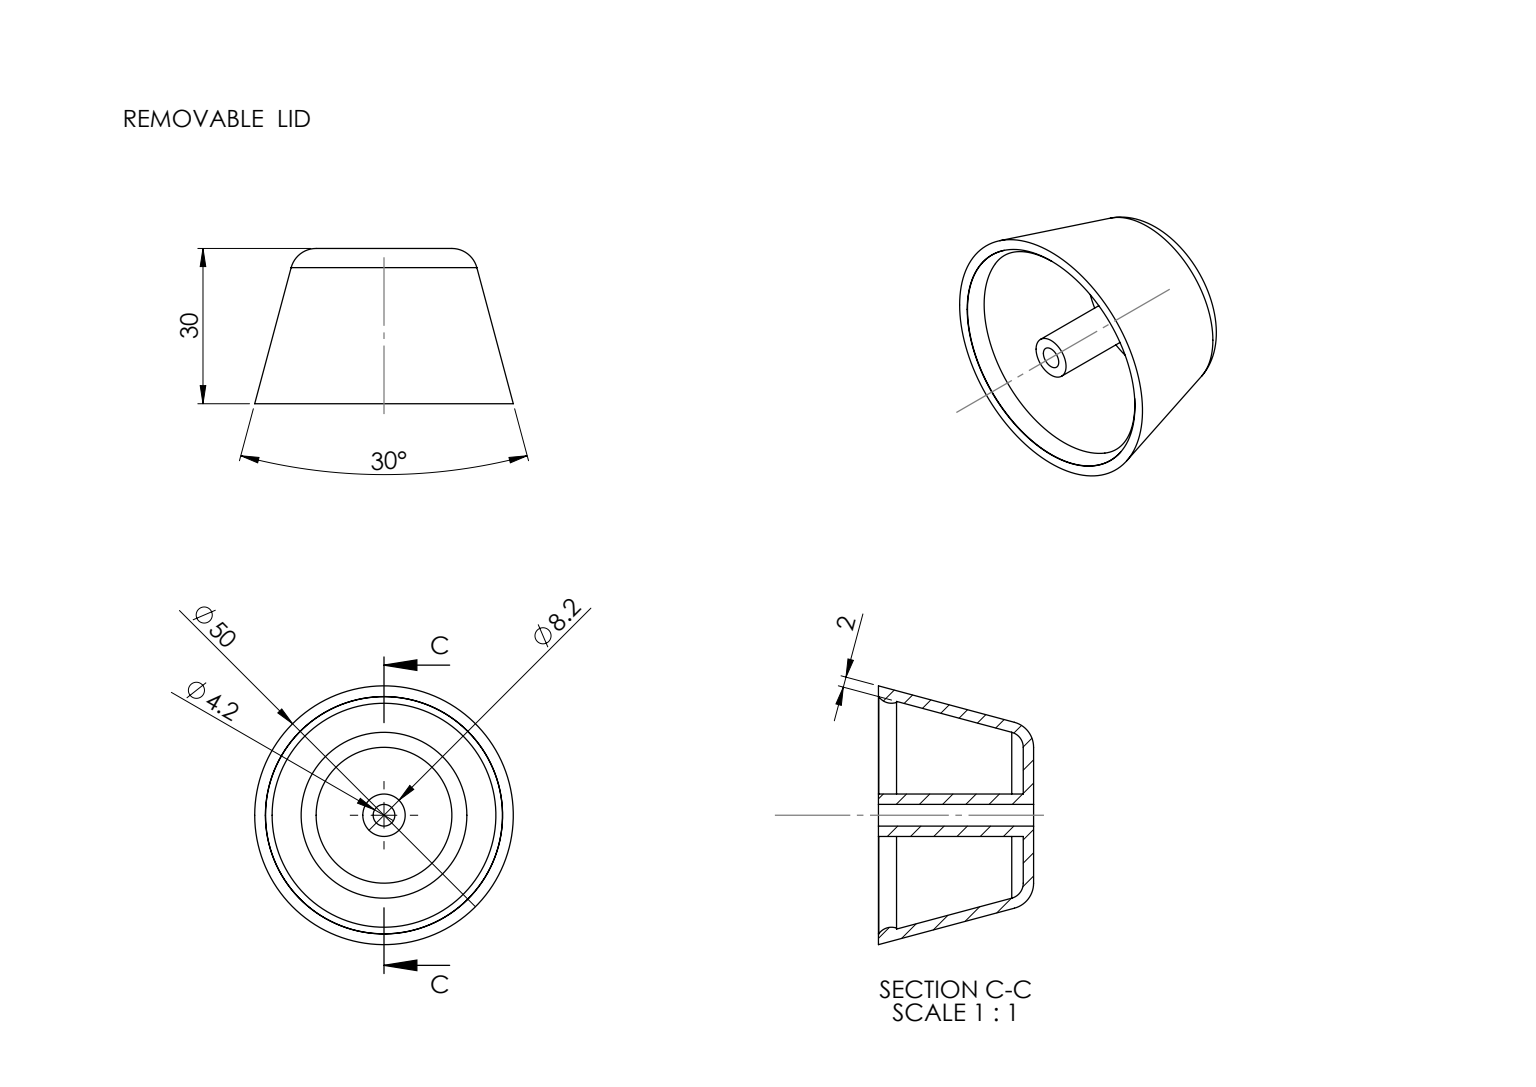
ISO-10303-21;
HEADER;
FILE_DESCRIPTION (('STEP AP214'),
    '1' );
FILE_NAME ('Removable  Lid.step',
    '2026-10-08T15:02:10',
    ( '' ),
    ( '' ),
    'SwSTEP 2.0',
    'SolidWorks 2026',
    '' );
FILE_SCHEMA (( 'AUTOMOTIVE_DESIGN' ));
ENDSEC;

DATA;
#102=ORIENTED_EDGE ( 'NONE', *, *, #14912, .T. ) ;
#167=ORIENTED_EDGE ( 'NONE', *, *, #18433, .F. ) ;
#184=DIRECTION ( 'NONE',  ( 0.000000000000000000, 0.000000000000000000, -1.000000000000000000 ) ) ;
#186=ADVANCED_FACE ( 'NONE', ( #19627 ), #432, .T. ) ;
#199=LINE ( 'NONE', #7182, #5891 ) ;
#273=EDGE_CURVE ( 'NONE', #12453, #12432, #18177, .T. ) ;
#319=CIRCLE ( 'NONE', #11443, 13.12488928717151637 ) ;
#342=CARTESIAN_POINT ( 'NONE',  ( 4.100000000000000533, 0.000000000000000000, -103.0000000000000000 ) ) ;
#421=DIRECTION ( 'NONE',  ( -0.2588190451025213501, 0.000000000000000000, 0.9659258262890680902 ) ) ;
#432=CONICAL_SURFACE ( 'NONE', #4015, 25.00000000000001066, 0.2617993877991500740 ) ;
#469=CONICAL_SURFACE ( 'NONE', #7660, 23.06814834742187514, 0.2617993877991500740 ) ;
#543=ORIENTED_EDGE ( 'NONE', *, *, #7416, .T. ) ;
#607=DIRECTION ( 'NONE',  ( -0.000000000000000000, -0.000000000000000000, 1.000000000000000000 ) ) ;
#632=ORIENTED_EDGE ( 'NONE', *, *, #6211, .T. ) ;
#650=DIRECTION ( 'NONE',  ( 1.000000000000000000, 0.000000000000000000, 0.000000000000000000 ) ) ;
#656=PRODUCT_DEFINITION_CONTEXT ( 'detailed design', #16058, 'design' ) ;
#700=CARTESIAN_POINT ( 'NONE',  ( 21.63401512838748175, 0.000000000000000000, -77.51594804401857175 ) ) ;
#709=ORIENTED_EDGE ( 'NONE', *, *, #8052, .T. ) ;
#780=CIRCLE ( 'NONE', #11560, 22.91388766833460977 ) ;
#809=DIRECTION ( 'NONE',  ( 1.000000000000000000, 0.000000000000000000, 0.000000000000000000 ) ) ;
#849=AXIS2_PLACEMENT_3D ( 'NONE', #7181, #9308, #14163 ) ;
#893=ORIENTED_EDGE ( 'NONE', *, *, #15181, .F. ) ;
#939=PRODUCT_DEFINITION_FORMATION_WITH_SPECIFIED_SOURCE ( 'ANY', '', #16966, .NOT_KNOWN. ) ;
#971=EDGE_LOOP ( 'NONE', ( #14065, #167, #6463, #2530 ) ) ;
#989=EDGE_CURVE ( 'NONE', #18158, #1422, #13733, .T. ) ;
#1060=DIRECTION ( 'NONE',  ( -0.000000000000000000, -0.000000000000000000, 1.000000000000000000 ) ) ;
#1093=PLANE ( 'NONE',  #20973 ) ;
#1094=UNCERTAINTY_MEASURE_WITH_UNIT (LENGTH_MEASURE( 1.000000000000000082E-05 ), #8420, 'distance_accuracy_value', 'NONE');
#1100=DIRECTION ( 'NONE',  ( -0.000000000000000000, -0.000000000000000000, 1.000000000000000000 ) ) ;
#1105=DIRECTION ( 'NONE',  ( -0.000000000000000000, -0.000000000000000000, 1.000000000000000000 ) ) ;
#1127=DIRECTION ( 'NONE',  ( -1.000000000000000000, 0.000000000000000000, 0.000000000000000000 ) ) ;
#1148=AXIS2_PLACEMENT_3D ( 'NONE', #12886, #17854, #11310 ) ;
#1216=DIRECTION ( 'NONE',  ( 0.000000000000000000, 0.000000000000000000, -1.000000000000000000 ) ) ;
#1241=AXIS2_PLACEMENT_3D ( 'NONE', #3863, #17832, #14871 ) ;
#1266=VERTEX_POINT ( 'NONE', #12280 ) ;
#1273=AXIS2_PLACEMENT_3D ( 'NONE', #3060, #20052, #18498 ) ;
#1317=FACE_OUTER_BOUND ( 'NONE', #4433, .T. ) ;
#1368=CARTESIAN_POINT ( 'NONE',  ( 0.000000000000000000, 0.000000000000000000, -100.7764571353075524 ) ) ;
#1402=ORIENTED_EDGE ( 'NONE', *, *, #13977, .F. ) ;
#1422=VERTEX_POINT ( 'NONE', #7666 ) ;
#1430=PRESENTATION_STYLE_ASSIGNMENT (( #18544 ) ) ;
#1440=EDGE_CURVE ( 'NONE', #15541, #8028, #2581, .T. ) ;
#1476=ORIENTED_EDGE ( 'NONE', *, *, #15181, .T. ) ;
#1528=ORIENTED_EDGE ( 'NONE', *, *, #6345, .F. ) ;
#1540=CARTESIAN_POINT ( 'NONE',  ( 0.000000000000000000, 0.000000000000000000, -75.00000000000000000 ) ) ;
#1586=CARTESIAN_POINT ( 'NONE',  ( 16.02266676603872142, -2.327704065170765110E-15, -100.7764571353075524 ) ) ;
#1599=AXIS2_PLACEMENT_3D ( 'NONE', #21798, #1216, #5136 ) ;
#1629=EDGE_LOOP ( 'NONE', ( #4957, #10753, #10472, #18603 ) ) ;
#1646=EDGE_CURVE ( 'NONE', #19741, #19867, #11223, .T. ) ;
#1666=TOROIDAL_SURFACE ( 'NONE', #17127, 24.63401512838748530, 3.000000000000004441 ) ;
#1681=ORIENTED_EDGE ( 'NONE', *, *, #18966, .T. ) ;
#1731=DIRECTION ( 'NONE',  ( -1.000000000000000000, -1.224646799147353454E-16, 0.000000000000000000 ) ) ;
#1906=CARTESIAN_POINT ( 'NONE',  ( 0.000000000000000000, 0.000000000000000000, -77.51594804401857175 ) ) ;
#1996=CARTESIAN_POINT ( 'NONE',  ( 0.000000000000000000, 0.000000000000000000, -75.00000000000000000 ) ) ;
#2037=DIRECTION ( 'NONE',  ( -0.000000000000000000, -1.000000000000000000, -0.000000000000000000 ) ) ;
#2135=ORIENTED_EDGE ( 'NONE', *, *, #12683, .T. ) ;
#2230=EDGE_CURVE ( 'NONE', #9583, #1422, #18773, .T. ) ;
#2248=AXIS2_PLACEMENT_3D ( 'NONE', #5502, #17450, #10466 ) ;
#2286=CARTESIAN_POINT ( 'NONE',  ( 0.000000000000000000, 0.000000000000000000, -103.0000000000000000 ) ) ;
#2303=DIRECTION ( 'NONE',  ( 0.000000000000000000, 0.000000000000000000, -1.000000000000000000 ) ) ;
#2309=SHAPE_DEFINITION_REPRESENTATION ( #4914, #3834 ) ;
#2335=COLOUR_RGB ( '', 0.72549020, 0.75294118, 0.79215686) ;
#2376=DIRECTION ( 'NONE',  ( 1.000000000000000000, 0.000000000000000000, 0.000000000000000000 ) ) ;
#2399=EDGE_CURVE ( 'NONE', #7331, #8832, #5603, .T. ) ;
#2493=CARTESIAN_POINT ( 'NONE',  ( -22.92944763917984830, 0.000000000000000000, -75.00000000000000000 ) ) ;
#2502=ORIENTED_EDGE ( 'NONE', *, *, #21773, .T. ) ;
#2530=ORIENTED_EDGE ( 'NONE', *, *, #3918, .T. ) ;
#2572=ADVANCED_FACE ( 'NONE', ( #16081 ), #7420, .F. ) ;
#2581=LINE ( 'NONE', #14647, #4356 ) ;
#2587=DIRECTION ( 'NONE',  ( -1.000000000000000000, 0.000000000000000000, 0.000000000000000000 ) ) ;
#2594=AXIS2_PLACEMENT_3D ( 'NONE', #7560, #14652, #13066 ) ;
#2607=CIRCLE ( 'NONE', #5842, 2.999999999999999112 ) ;
#2707=DIRECTION ( 'NONE',  ( 1.000000000000000000, 0.000000000000000000, 0.000000000000000000 ) ) ;
#2721=VECTOR ( 'NONE', #421, 1000.000000000000000 ) ;
#2774=DIRECTION ( 'NONE',  ( -0.000000000000000000, -0.000000000000000000, 1.000000000000000000 ) ) ;
#2867=VERTEX_POINT ( 'NONE', #14502 ) ;
#2990=CYLINDRICAL_SURFACE ( 'NONE', #10486, 2.100000000000000089 ) ;
#2992=LINE ( 'NONE', #4575, #19523 ) ;
#3044=FACE_OUTER_BOUND ( 'NONE', #15970, .T. ) ;
#3060=CARTESIAN_POINT ( 'NONE',  ( 0.000000000000000000, 0.000000000000000000, -101.2940952255125922 ) ) ;
#3096=CIRCLE ( 'NONE', #11018, 25.00000000000001066 ) ;
#3108=DIRECTION ( 'NONE',  ( -1.000000000000000000, 0.000000000000000000, -0.000000000000000000 ) ) ;
#3156=EDGE_CURVE ( 'NONE', #9492, #8832, #20066, .T. ) ;
#3240=VERTEX_POINT ( 'NONE', #4340 ) ;
#3250=FACE_OUTER_BOUND ( 'NONE', #12502, .T. ) ;
#3256=DIRECTION ( 'NONE',  ( -1.000000000000000000, 0.000000000000000000, 0.000000000000000000 ) ) ;
#3264=EDGE_LOOP ( 'NONE', ( #19648, #10645 ) ) ;
#3283=DIRECTION ( 'NONE',  ( 0.000000000000000000, 0.000000000000000000, -1.000000000000000000 ) ) ;
#3352=ORIENTED_EDGE ( 'NONE', *, *, #2399, .T. ) ;
#3385=DIRECTION ( 'NONE',  ( 0.000000000000000000, 0.000000000000000000, -1.000000000000000000 ) ) ;
#3417=ORIENTED_EDGE ( 'NONE', *, *, #12728, .T. ) ;
#3431=VERTEX_POINT ( 'NONE', #9869 ) ;
#3447=ADVANCED_FACE ( 'NONE', ( #8186 ), #19357, .T. ) ;
#3549=ORIENTED_EDGE ( 'NONE', *, *, #3744, .T. ) ;
#3577=CARTESIAN_POINT ( 'NONE',  ( 23.06814834742187514, -2.825033403592650701E-15, -74.48236190979496030 ) ) ;
#3589=DIRECTION ( 'NONE',  ( -0.000000000000000000, -0.000000000000000000, 1.000000000000000000 ) ) ;
#3687=TOROIDAL_SURFACE ( 'NONE', #6567, 24.63401512838748530, 3.000000000000004441 ) ;
#3744=EDGE_CURVE ( 'NONE', #17843, #1266, #319, .T. ) ;
#3749=ORIENTED_EDGE ( 'NONE', *, *, #4848, .T. ) ;
#3774=AXIS2_PLACEMENT_3D ( 'NONE', #4834, #4714, #16779 ) ;
#3780=ORIENTED_EDGE ( 'NONE', *, *, #989, .F. ) ;
#3834=SHAPE_REPRESENTATION ( 'Removable  Lid', ( #6677 ), #10599 ) ;
#3863=CARTESIAN_POINT ( 'NONE',  ( 0.000000000000000000, 0.000000000000000000, -75.00000000000000000 ) ) ;
#3878=CARTESIAN_POINT ( 'NONE',  ( 4.100000000000000533, 0.000000000000000000, -75.00000000000000000 ) ) ;
#3918=EDGE_CURVE ( 'NONE', #7331, #9583, #9301, .T. ) ;
#3924=DIRECTION ( 'NONE',  ( -1.000000000000000000, 0.000000000000000000, -0.000000000000000000 ) ) ;
#3966=CIRCLE ( 'NONE', #19425, 13.12488928717151637 ) ;
#4008=DIRECTION ( 'NONE',  ( -1.000000000000000000, 0.000000000000000000, 0.000000000000000000 ) ) ;
#4015=AXIS2_PLACEMENT_3D ( 'NONE', #21200, #5574, #10760 ) ;
#4088=AXIS2_PLACEMENT_3D ( 'NONE', #16522, #1100, #13367 ) ;
#4133=VERTEX_POINT ( 'NONE', #3878 ) ;
#4134=( GEOMETRIC_REPRESENTATION_CONTEXT ( 3 ) GLOBAL_UNCERTAINTY_ASSIGNED_CONTEXT ( ( #12593 ) ) GLOBAL_UNIT_ASSIGNED_CONTEXT ( ( #18657, #15061, #6726 ) ) REPRESENTATION_CONTEXT ( 'NONE', 'WORKASPACE' ) );
#4153=EDGE_LOOP ( 'NONE', ( #13725, #3352, #15634, #8574 ) ) ;
#4176=LINE ( 'NONE', #10938, #19976 ) ;
#4210=FACE_BOUND ( 'NONE', #14141, .T. ) ;
#4249=AXIS2_PLACEMENT_3D ( 'NONE', #17517, #15827, #184 ) ;
#4316=DIRECTION ( 'NONE',  ( -1.000000000000000000, 0.000000000000000000, 0.000000000000000000 ) ) ;
#4325=FACE_BOUND ( 'NONE', #5598, .T. ) ;
#4335=ORIENTED_EDGE ( 'NONE', *, *, #7895, .F. ) ;
#4340=CARTESIAN_POINT ( 'NONE',  ( 25.00000000000001066, -3.061616997868384226E-15, -75.00000000000000000 ) ) ;
#4356=VECTOR ( 'NONE', #12727, 1000.000000000000000 ) ;
#4385=DIRECTION ( 'NONE',  ( -0.000000000000000000, -0.000000000000000000, 1.000000000000000000 ) ) ;
#4412=FILL_AREA_STYLE ('',( #16363 ) ) ;
#4427=DIRECTION ( 'NONE',  ( 0.000000000000000000, 0.000000000000000000, -1.000000000000000000 ) ) ;
#4433=EDGE_LOOP ( 'NONE', ( #1402, #5404, #7386, #10652 ) ) ;
#4521=ADVANCED_FACE ( 'NONE', ( #4210, #21637 ), #16260, .F. ) ;
#4553=CARTESIAN_POINT ( 'NONE',  ( 4.100000000000000533, 0.000000000000000000, -126.0000000000000284 ) ) ;
#4575=CARTESIAN_POINT ( 'NONE',  ( 25.00000000000001066, -3.061616997868384226E-15, -75.00000000000000000 ) ) ;
#4661=DIRECTION ( 'NONE',  ( -0.000000000000000000, -0.000000000000000000, 1.000000000000000000 ) ) ;
#4714=DIRECTION ( 'NONE',  ( 0.000000000000000000, 0.000000000000000000, -1.000000000000000000 ) ) ;
#4732=DIRECTION ( 'NONE',  ( -0.000000000000000000, -0.000000000000000000, 1.000000000000000000 ) ) ;
#4795=DIRECTION ( 'NONE',  ( -1.000000000000000000, 0.000000000000000000, 0.000000000000000000 ) ) ;
#4828=APPLICATION_CONTEXT ( 'automotive_design' ) ;
#4830=AXIS2_PLACEMENT_3D ( 'NONE', #2286, #607, #1127 ) ;
#4834=CARTESIAN_POINT ( 'NONE',  ( 0.000000000000000000, 0.000000000000000000, -75.00000000000000000 ) ) ;
#4848=EDGE_CURVE ( 'NONE', #1422, #18158, #15892, .T. ) ;
#4866=AXIS2_PLACEMENT_3D ( 'NONE', #11626, #13095, #12979 ) ;
#4914=PRODUCT_DEFINITION_SHAPE ( 'NONE', 'NONE',  #14016 ) ;
#4921=DIRECTION ( 'NONE',  ( -1.000000000000000000, 0.000000000000000000, 0.000000000000000000 ) ) ;
#4957=ORIENTED_EDGE ( 'NONE', *, *, #9109, .F. ) ;
#5039=ORIENTED_EDGE ( 'NONE', *, *, #273, .F. ) ;
#5055=CARTESIAN_POINT ( 'NONE',  ( 0.000000000000000000, 0.000000000000000000, -105.0000000000000000 ) ) ;
#5056=FACE_OUTER_BOUND ( 'NONE', #16912, .T. ) ;
#5087=VECTOR ( 'NONE', #1060, 1000.000000000000000 ) ;
#5136=DIRECTION ( 'NONE',  ( -1.000000000000000000, 0.000000000000000000, 0.000000000000000000 ) ) ;
#5161=CIRCLE ( 'NONE', #4088, 17.95451841861686049 ) ;
#5248=CIRCLE ( 'NONE', #17491, 2.100000000000000089 ) ;
#5273=FACE_OUTER_BOUND ( 'NONE', #16255, .T. ) ;
#5370=ORIENTED_EDGE ( 'NONE', *, *, #6806, .T. ) ;
#5396=ADVANCED_FACE ( 'NONE', ( #1317 ), #2990, .F. ) ;
#5404=ORIENTED_EDGE ( 'NONE', *, *, #21485, .F. ) ;
#5496=EDGE_CURVE ( 'NONE', #7331, #6505, #780, .T. ) ;
#5501=CARTESIAN_POINT ( 'NONE',  ( 2.100000000000000089, 0.000000000000000000, -105.0000000000000000 ) ) ;
#5502=CARTESIAN_POINT ( 'NONE',  ( 0.000000000000000000, 0.000000000000000000, -77.51594804401857175 ) ) ;
#5541=AXIS2_PLACEMENT_3D ( 'NONE', #22024, #6733, #4921 ) ;
#5557=CIRCLE ( 'NONE', #13114, 5.000000000000004441 ) ;
#5574=DIRECTION ( 'NONE',  ( -0.000000000000000000, -0.000000000000000000, 1.000000000000000000 ) ) ;
#5580=CIRCLE ( 'NONE', #18165, 3.000000000000006217 ) ;
#5595=FACE_OUTER_BOUND ( 'NONE', #4153, .T. ) ;
#5598=EDGE_LOOP ( 'NONE', ( #9277, #10311 ) ) ;
#5603=LINE ( 'NONE', #3577, #11109 ) ;
#5617=CARTESIAN_POINT ( 'NONE',  ( -17.95451841861686049, 0.000000000000000000, -101.2940952255125922 ) ) ;
#5643=FACE_OUTER_BOUND ( 'NONE', #971, .T. ) ;
#5664=DIRECTION ( 'NONE',  ( 0.000000000000000000, 0.000000000000000000, -1.000000000000000000 ) ) ;
#5710=DIRECTION ( 'NONE',  ( 0.2588190451025213501, -3.169619151431772337E-17, 0.9659258262890680902 ) ) ;
#5788=VERTEX_POINT ( 'NONE', #10867 ) ;
#5804=AXIS2_PLACEMENT_3D ( 'NONE', #11415, #2303, #9187 ) ;
#5842=AXIS2_PLACEMENT_3D ( 'NONE', #11755, #17155, #1731 ) ;
#5891=VECTOR ( 'NONE', #13827, 1000.000000000000000 ) ;
#5905=CARTESIAN_POINT ( 'NONE',  ( 0.000000000000000000, 0.000000000000000000, -105.0000000000000000 ) ) ;
#5909=CIRCLE ( 'NONE', #4830, 4.100000000000000533 ) ;
#5914=CARTESIAN_POINT ( 'NONE',  ( 13.12488928717151637, 1.784773061176598909E-15, -103.0000000000000000 ) ) ;
#5918=DIRECTION ( 'NONE',  ( 0.000000000000000000, 0.000000000000000000, -1.000000000000000000 ) ) ;
#5922=CARTESIAN_POINT ( 'NONE',  ( 0.000000000000000000, 0.000000000000000000, -74.48236190979496030 ) ) ;
#5970=CARTESIAN_POINT ( 'NONE',  ( 0.000000000000000000, 0.000000000000000000, -74.48236190979496030 ) ) ;
#6000=SURFACE_STYLE_FILL_AREA ( #4412 ) ;
#6031=CARTESIAN_POINT ( 'NONE',  ( 22.92944763917984830, -2.808047465753843770E-15, -75.00000000000000000 ) ) ;
#6067=EDGE_CURVE ( 'NONE', #5788, #2867, #15536, .T. ) ;
#6100=ORIENTED_EDGE ( 'NONE', *, *, #22062, .F. ) ;
#6187=DIRECTION ( 'NONE',  ( -0.000000000000000000, -0.000000000000000000, 1.000000000000000000 ) ) ;
#6211=EDGE_CURVE ( 'NONE', #2867, #3431, #3966, .T. ) ;
#6245=CARTESIAN_POINT ( 'NONE',  ( -21.80000000000000071, 2.669730022141230095E-15, -78.50000000000000000 ) ) ;
#6345=EDGE_CURVE ( 'NONE', #8548, #1266, #17690, .T. ) ;
#6366=ORIENTED_EDGE ( 'NONE', *, *, #21188, .F. ) ;
#6377=FACE_OUTER_BOUND ( 'NONE', #21008, .T. ) ;
#6413=DIRECTION ( 'NONE',  ( 1.000000000000000000, 0.000000000000000000, 0.000000000000000000 ) ) ;
#6418=CARTESIAN_POINT ( 'NONE',  ( 0.000000000000000000, 0.000000000000000000, -75.00000000000000000 ) ) ;
#6463=ORIENTED_EDGE ( 'NONE', *, *, #22062, .T. ) ;
#6482=ORIENTED_EDGE ( 'NONE', *, *, #1646, .T. ) ;
#6489=FILL_AREA_STYLE_COLOUR ( '', #2335 ) ;
#6501=CYLINDRICAL_SURFACE ( 'NONE', #19856, 4.100000000000000533 ) ;
#6505=VERTEX_POINT ( 'NONE', #21792 ) ;
#6542=CARTESIAN_POINT ( 'NONE',  ( 0.000000000000000000, 0.000000000000000000, -74.48236190979496030 ) ) ;
#6550=TOROIDAL_SURFACE ( 'NONE', #2248, 24.63401512838748530, 3.000000000000004441 ) ;
#6566=DIRECTION ( 'NONE',  ( -0.000000000000000000, -0.000000000000000000, 1.000000000000000000 ) ) ;
#6567=AXIS2_PLACEMENT_3D ( 'NONE', #9269, #17707, #809 ) ;
#6628=AXIS2_PLACEMENT_3D ( 'NONE', #18664, #22142, #22249 ) ;
#6677=AXIS2_PLACEMENT_3D ( 'NONE', #18028, #16226, #2707 ) ;
#6712=ORIENTED_EDGE ( 'NONE', *, *, #14581, .F. ) ;
#6726=( NAMED_UNIT ( * ) SI_UNIT ( $, .STERADIAN. ) SOLID_ANGLE_UNIT ( ) );
#6733=DIRECTION ( 'NONE',  ( -0.000000000000000000, -0.000000000000000000, 1.000000000000000000 ) ) ;
#6806=EDGE_CURVE ( 'NONE', #6505, #9492, #8981, .T. ) ;
#6828=EDGE_CURVE ( 'NONE', #8028, #3240, #14260, .T. ) ;
#6880=EDGE_LOOP ( 'NONE', ( #22032, #6100, #5370, #893 ) ) ;
#6997=FACE_OUTER_BOUND ( 'NONE', #15192, .T. ) ;
#7013=DIRECTION ( 'NONE',  ( -0.000000000000000000, -0.000000000000000000, 1.000000000000000000 ) ) ;
#7049=ORIENTED_EDGE ( 'NONE', *, *, #6067, .T. ) ;
#7114=DIRECTION ( 'NONE',  ( 1.000000000000000000, 0.000000000000000000, 0.000000000000000000 ) ) ;
#7129=DIRECTION ( 'NONE',  ( -0.000000000000000000, -0.000000000000000000, 1.000000000000000000 ) ) ;
#7181=CARTESIAN_POINT ( 'NONE',  ( 0.000000000000000000, 0.000000000000000000, -99.99999999999998579 ) ) ;
#7182=CARTESIAN_POINT ( 'NONE',  ( 23.06814834742187514, -2.825033403592650701E-15, -74.48236190979496030 ) ) ;
#7279=ORIENTED_EDGE ( 'NONE', *, *, #14581, .T. ) ;
#7331=VERTEX_POINT ( 'NONE', #19262 ) ;
#7367=ADVANCED_FACE ( 'NONE', ( #5643 ), #1666, .T. ) ;
#7375=CARTESIAN_POINT ( 'NONE',  ( -13.12488928717151637, 0.000000000000000000, -99.99999999999998579 ) ) ;
#7386=ORIENTED_EDGE ( 'NONE', *, *, #9658, .T. ) ;
#7416=EDGE_CURVE ( 'NONE', #8548, #19867, #4176, .T. ) ;
#7420=CYLINDRICAL_SURFACE ( 'NONE', #20796, 2.100000000000000089 ) ;
#7476=ORIENTED_EDGE ( 'NONE', *, *, #12728, .F. ) ;
#7547=ORIENTED_EDGE ( 'NONE', *, *, #21773, .F. ) ;
#7560=CARTESIAN_POINT ( 'NONE',  ( -24.63401512838748530, 3.016796777712720900E-15, -77.51594804401857175 ) ) ;
#7566=CARTESIAN_POINT ( 'NONE',  ( 0.000000000000000000, 0.000000000000000000, -77.51594804401857175 ) ) ;
#7634=EDGE_LOOP ( 'NONE', ( #10379, #8677, #102, #18423 ) ) ;
#7659=CARTESIAN_POINT ( 'NONE',  ( 0.000000000000000000, 0.000000000000000000, -78.50000000000000000 ) ) ;
#7660=AXIS2_PLACEMENT_3D ( 'NONE', #5922, #19322, #17760 ) ;
#7666=CARTESIAN_POINT ( 'NONE',  ( 21.80000000000000071, 0.000000000000000000, -78.50000000000000000 ) ) ;
#7674=FACE_OUTER_BOUND ( 'NONE', #6880, .T. ) ;
#7704=CARTESIAN_POINT ( 'NONE',  ( -2.100000000000000089, 2.571758278209441957E-16, -75.00000000000000000 ) ) ;
#7747=STYLED_ITEM ( 'NONE', ( #1430 ), #13667 ) ;
#7780=CIRCLE ( 'NONE', #16377, 22.91388766833460977 ) ;
#7835=ORIENTED_EDGE ( 'NONE', *, *, #12683, .F. ) ;
#7880=VERTEX_POINT ( 'NONE', #1586 ) ;
#7888=EDGE_CURVE ( 'NONE', #12432, #4133, #17849, .T. ) ;
#7895=EDGE_CURVE ( 'NONE', #13423, #21223, #5248, .T. ) ;
#7923=( NAMED_UNIT ( * ) PLANE_ANGLE_UNIT ( ) SI_UNIT ( $, .RADIAN. ) );
#7980=CARTESIAN_POINT ( 'NONE',  ( 21.99162546567091425, -2.693197373458130478E-15, -78.50000000000000000 ) ) ;
#8028=VERTEX_POINT ( 'NONE', #11936 ) ;
#8030=EDGE_LOOP ( 'NONE', ( #8652, #17878, #709, #21956 ) ) ;
#8052=EDGE_CURVE ( 'NONE', #3240, #8028, #3096, .T. ) ;
#8062=DIRECTION ( 'NONE',  ( -1.000000000000000000, 0.000000000000000000, -0.000000000000000000 ) ) ;
#8063=AXIS2_PLACEMENT_3D ( 'NONE', #18520, #10077, #8062 ) ;
#8078=DIRECTION ( 'NONE',  ( 0.000000000000000000, 0.000000000000000000, -1.000000000000000000 ) ) ;
#8186=FACE_OUTER_BOUND ( 'NONE', #13352, .T. ) ;
#8266=CARTESIAN_POINT ( 'NONE',  ( 0.000000000000000000, 0.000000000000000000, -78.50000000000000000 ) ) ;
#8295=CARTESIAN_POINT ( 'NONE',  ( 0.000000000000000000, 0.000000000000000000, -103.0000000000000000 ) ) ;
#8310=FACE_OUTER_BOUND ( 'NONE', #1629, .T. ) ;
#8352=EDGE_LOOP ( 'NONE', ( #17790, #9423, #3549, #1528 ) ) ;
#8420=( LENGTH_UNIT ( ) NAMED_UNIT ( * ) SI_UNIT ( .MILLI., .METRE. ) );
#8491=DIRECTION ( 'NONE',  ( -1.000000000000000000, 1.224646799147352961E-16, 0.000000000000000000 ) ) ;
#8525=DIRECTION ( 'NONE',  ( 0.000000000000000000, 0.000000000000000000, -1.000000000000000000 ) ) ;
#8548=VERTEX_POINT ( 'NONE', #12360 ) ;
#8574=ORIENTED_EDGE ( 'NONE', *, *, #6806, .F. ) ;
#8578=ADVANCED_FACE ( 'NONE', ( #15849 ), #11110, .T. ) ;
#8611=ADVANCED_FACE ( 'NONE', ( #5595 ), #17350, .F. ) ;
#8632=ORIENTED_EDGE ( 'NONE', *, *, #14777, .F. ) ;
#8652=ORIENTED_EDGE ( 'NONE', *, *, #12559, .T. ) ;
#8663=ADVANCED_FACE ( 'NONE', ( #12688 ), #469, .F. ) ;
#8677=ORIENTED_EDGE ( 'NONE', *, *, #12559, .F. ) ;
#8711=CIRCLE ( 'NONE', #14838, 13.12488928717151637 ) ;
#8722=EDGE_LOOP ( 'NONE', ( #7547, #13016, #10974, #3780 ) ) ;
#8832=VERTEX_POINT ( 'NONE', #6031 ) ;
#8834=AXIS2_PLACEMENT_3D ( 'NONE', #22202, #7013, #12186 ) ;
#8865=ORIENTED_EDGE ( 'NONE', *, *, #13977, .T. ) ;
#8877=CARTESIAN_POINT ( 'NONE',  ( 0.000000000000000000, 0.000000000000000000, -75.00000000000000000 ) ) ;
#8899=DIRECTION ( 'NONE',  ( -1.000000000000000000, 0.000000000000000000, 0.000000000000000000 ) ) ;
#8941=AXIS2_PLACEMENT_3D ( 'NONE', #11336, #8078, #17986 ) ;
#8974=ORIENTED_EDGE ( 'NONE', *, *, #5496, .T. ) ;
#8981=LINE ( 'NONE', #14488, #2721 ) ;
#9088=DIRECTION ( 'NONE',  ( -1.000000000000000000, 0.000000000000000000, 0.000000000000000000 ) ) ;
#9108=CIRCLE ( 'NONE', #21657, 16.02266676603872142 ) ;
#9109=EDGE_CURVE ( 'NONE', #7880, #17843, #2607, .T. ) ;
#9136=CONICAL_SURFACE ( 'NONE', #19889, 25.00000000000001066, 0.2617993877991500740 ) ;
#9187=DIRECTION ( 'NONE',  ( -1.000000000000000000, 0.000000000000000000, -0.000000000000000000 ) ) ;
#9188=ORIENTED_EDGE ( 'NONE', *, *, #3918, .F. ) ;
#9225=AXIS2_PLACEMENT_3D ( 'NONE', #17756, #5918, #9088 ) ;
#9269=CARTESIAN_POINT ( 'NONE',  ( 0.000000000000000000, 0.000000000000000000, -77.51594804401857175 ) ) ;
#9277=ORIENTED_EDGE ( 'NONE', *, *, #21485, .T. ) ;
#9301=CIRCLE ( 'NONE', #4249, 3.000000000000002665 ) ;
#9305=ORIENTED_EDGE ( 'NONE', *, *, #12993, .T. ) ;
#9308=DIRECTION ( 'NONE',  ( 0.000000000000000000, 0.000000000000000000, -1.000000000000000000 ) ) ;
#9309=CARTESIAN_POINT ( 'NONE',  ( 2.100000000000000089, 0.000000000000000000, -75.00000000000000000 ) ) ;
#9346=ORIENTED_EDGE ( 'NONE', *, *, #7888, .T. ) ;
#9365=DIRECTION ( 'NONE',  ( -0.2588190451025213501, 0.000000000000000000, 0.9659258262890680902 ) ) ;
#9373=FACE_OUTER_BOUND ( 'NONE', #8722, .T. ) ;
#9418=ADVANCED_FACE ( 'NONE', ( #9373 ), #3687, .T. ) ;
#9423=ORIENTED_EDGE ( 'NONE', *, *, #9109, .T. ) ;
#9492=VERTEX_POINT ( 'NONE', #2493 ) ;
#9507=ORIENTED_EDGE ( 'NONE', *, *, #9879, .F. ) ;
#9559=AXIS2_PLACEMENT_3D ( 'NONE', #22088, #3283, #15355 ) ;
#9583=VERTEX_POINT ( 'NONE', #700 ) ;
#9621=CARTESIAN_POINT ( 'NONE',  ( -4.100000000000000533, 5.021051876504148371E-16, -126.0000000000000284 ) ) ;
#9658=EDGE_CURVE ( 'NONE', #15704, #13423, #21277, .T. ) ;
#9741=PLANE ( 'NONE',  #8063 ) ;
#9869=CARTESIAN_POINT ( 'NONE',  ( -13.12488928717151637, 0.000000000000000000, -105.0000000000000000 ) ) ;
#9873=CARTESIAN_POINT ( 'NONE',  ( 0.000000000000000000, 0.000000000000000000, -126.0000000000000284 ) ) ;
#9874=CIRCLE ( 'NONE', #1241, 4.100000000000000533 ) ;
#9879=EDGE_CURVE ( 'NONE', #7880, #8548, #9108, .T. ) ;
#9907=ADVANCED_FACE ( 'NONE', ( #3044, #14667 ), #21727, .F. ) ;
#9917=FACE_OUTER_BOUND ( 'NONE', #7634, .T. ) ;
#9989=DIRECTION ( 'NONE',  ( -0.000000000000000000, -0.000000000000000000, 1.000000000000000000 ) ) ;
#10002=DIRECTION ( 'NONE',  ( -0.000000000000000000, -0.000000000000000000, 1.000000000000000000 ) ) ;
#10077=DIRECTION ( 'NONE',  ( 0.000000000000000000, 0.000000000000000000, -1.000000000000000000 ) ) ;
#10097=CARTESIAN_POINT ( 'NONE',  ( 0.000000000000000000, 0.000000000000000000, -75.05807060175870049 ) ) ;
#10204=DIRECTION ( 'NONE',  ( -1.000000000000000000, 0.000000000000000000, 0.000000000000000000 ) ) ;
#10259=EDGE_LOOP ( 'NONE', ( #12552, #632 ) ) ;
#10311=ORIENTED_EDGE ( 'NONE', *, *, #15458, .T. ) ;
#10379=ORIENTED_EDGE ( 'NONE', *, *, #6067, .F. ) ;
#10381=ADVANCED_FACE ( 'NONE', ( #6997 ), #20580, .F. ) ;
#10466=DIRECTION ( 'NONE',  ( 1.000000000000000000, 0.000000000000000000, 0.000000000000000000 ) ) ;
#10472=ORIENTED_EDGE ( 'NONE', *, *, #6345, .T. ) ;
#10478=DIRECTION ( 'NONE',  ( 1.000000000000000000, 0.000000000000000000, 0.000000000000000000 ) ) ;
#10486=AXIS2_PLACEMENT_3D ( 'NONE', #9873, #17075, #16739 ) ;
#10508=CIRCLE ( 'NONE', #2594, 3.000000000000006217 ) ;
#10567=TOROIDAL_SURFACE ( 'NONE', #849, 13.12488928717151637, 3.000000000000000000 ) ;
#10599=( GEOMETRIC_REPRESENTATION_CONTEXT ( 3 ) GLOBAL_UNCERTAINTY_ASSIGNED_CONTEXT ( ( #1094 ) ) GLOBAL_UNIT_ASSIGNED_CONTEXT ( ( #8420, #22137, #12011 ) ) REPRESENTATION_CONTEXT ( 'NONE', 'WORKASPACE' ) );
#10617=MECHANICAL_DESIGN_GEOMETRIC_PRESENTATION_REPRESENTATION('',(#7747),#4134);
#10645=ORIENTED_EDGE ( 'NONE', *, *, #3744, .F. ) ;
#10652=ORIENTED_EDGE ( 'NONE', *, *, #7895, .T. ) ;
#10753=ORIENTED_EDGE ( 'NONE', *, *, #9879, .T. ) ;
#10760=DIRECTION ( 'NONE',  ( -1.000000000000000000, 0.000000000000000000, 0.000000000000000000 ) ) ;
#10856=EDGE_LOOP ( 'NONE', ( #14828, #8865, #3417, #11068 ) ) ;
#10867=CARTESIAN_POINT ( 'NONE',  ( 17.95451841861686049, -2.630205674513758549E-15, -101.2940952255125922 ) ) ;
#10872=ORIENTED_EDGE ( 'NONE', *, *, #21188, .T. ) ;
#10891=ORIENTED_EDGE ( 'NONE', *, *, #11148, .F. ) ;
#10899=AXIS2_PLACEMENT_3D ( 'NONE', #6542, #12064, #13413 ) ;
#10938=CARTESIAN_POINT ( 'NONE',  ( -23.06814834742187514, 0.000000000000000000, -74.48236190979496030 ) ) ;
#10974=ORIENTED_EDGE ( 'NONE', *, *, #2230, .T. ) ;
#11007=ORIENTED_EDGE ( 'NONE', *, *, #14912, .F. ) ;
#11018=AXIS2_PLACEMENT_3D ( 'NONE', #8877, #15741, #19095 ) ;
#11068=ORIENTED_EDGE ( 'NONE', *, *, #9658, .F. ) ;
#11071=ADVANCED_FACE ( 'NONE', ( #6377 ), #9136, .T. ) ;
#11109=VECTOR ( 'NONE', #5710, 1000.000000000000000 ) ;
#11110=CYLINDRICAL_SURFACE ( 'NONE', #16278, 4.100000000000000533 ) ;
#11148=EDGE_CURVE ( 'NONE', #5788, #3240, #2992, .T. ) ;
#11168=DIRECTION ( 'NONE',  ( -1.000000000000000000, 0.000000000000000000, -0.000000000000000000 ) ) ;
#11184=( LENGTH_UNIT ( ) NAMED_UNIT ( * ) SI_UNIT ( .MILLI., .METRE. ) );
#11223=CIRCLE ( 'NONE', #11948, 21.99162546567091070 ) ;
#11272=ADVANCED_FACE ( 'NONE', ( #21790, #21899 ), #1093, .F. ) ;
#11295=SURFACE_STYLE_USAGE ( .BOTH. , #13207 ) ;
#11310=DIRECTION ( 'NONE',  ( -1.000000000000000000, -1.224646799147352961E-16, 0.000000000000000000 ) ) ;
#11336=CARTESIAN_POINT ( 'NONE',  ( 0.000000000000000000, 0.000000000000000000, -75.00000000000000000 ) ) ;
#11415=CARTESIAN_POINT ( 'NONE',  ( 0.000000000000000000, 0.000000000000000000, -103.0000000000000000 ) ) ;
#11443=AXIS2_PLACEMENT_3D ( 'NONE', #8295, #8525, #11783 ) ;
#11560=AXIS2_PLACEMENT_3D ( 'NONE', #10097, #9989, #22133 ) ;
#11597=AXIS2_PLACEMENT_3D ( 'NONE', #12476, #16072, #4008 ) ;
#11626=CARTESIAN_POINT ( 'NONE',  ( 0.000000000000000000, 0.000000000000000000, -78.50000000000000000 ) ) ;
#11648=FACE_OUTER_BOUND ( 'NONE', #10259, .T. ) ;
#11671=CARTESIAN_POINT ( 'NONE',  ( 0.000000000000000000, 0.000000000000000000, -75.00000000000000000 ) ) ;
#11755=CARTESIAN_POINT ( 'NONE',  ( 13.12488928717151637, 1.607335365469798272E-15, -99.99999999999998579 ) ) ;
#11768=CARTESIAN_POINT ( 'NONE',  ( -2.100000000000000089, 2.571758278209441957E-16, -126.0000000000000284 ) ) ;
#11783=DIRECTION ( 'NONE',  ( -1.000000000000000000, 0.000000000000000000, 0.000000000000000000 ) ) ;
#11873=LINE ( 'NONE', #4553, #12382 ) ;
#11931=DIRECTION ( 'NONE',  ( -0.000000000000000000, -0.000000000000000000, 1.000000000000000000 ) ) ;
#11936=CARTESIAN_POINT ( 'NONE',  ( -25.00000000000001066, 0.000000000000000000, -75.00000000000000000 ) ) ;
#11948=AXIS2_PLACEMENT_3D ( 'NONE', #7659, #21698, #21365 ) ;
#12011=( NAMED_UNIT ( * ) SI_UNIT ( $, .STERADIAN. ) SOLID_ANGLE_UNIT ( ) );
#12013=CIRCLE ( 'NONE', #6628, 2.100000000000000089 ) ;
#12026=ORIENTED_EDGE ( 'NONE', *, *, #4848, .F. ) ;
#12042=CIRCLE ( 'NONE', #3774, 22.92944763917984474 ) ;
#12063=( GEOMETRIC_REPRESENTATION_CONTEXT ( 3 ) GLOBAL_UNCERTAINTY_ASSIGNED_CONTEXT ( ( #21791 ) ) GLOBAL_UNIT_ASSIGNED_CONTEXT ( ( #11184, #7923, #19722 ) ) REPRESENTATION_CONTEXT ( 'NONE', 'WORKASPACE' ) );
#12064=DIRECTION ( 'NONE',  ( -0.000000000000000000, -0.000000000000000000, 1.000000000000000000 ) ) ;
#12154=PLANE ( 'NONE',  #19939 ) ;
#12170=CARTESIAN_POINT ( 'NONE',  ( 0.000000000000000000, 0.000000000000000000, -78.50000000000000000 ) ) ;
#12186=DIRECTION ( 'NONE',  ( -1.000000000000000000, 0.000000000000000000, 0.000000000000000000 ) ) ;
#12253=DIRECTION ( 'NONE',  ( 0.000000000000000000, -1.000000000000000000, 0.000000000000000000 ) ) ;
#12280=CARTESIAN_POINT ( 'NONE',  ( -13.12488928717151637, 0.000000000000000000, -103.0000000000000000 ) ) ;
#12360=CARTESIAN_POINT ( 'NONE',  ( -16.02266676603872142, 0.000000000000000000, -100.7764571353075524 ) ) ;
#12382=VECTOR ( 'NONE', #16828, 1000.000000000000000 ) ;
#12419=MECHANICAL_DESIGN_GEOMETRIC_PRESENTATION_REPRESENTATION('',(#17096),#12063);
#12432=VERTEX_POINT ( 'NONE', #16305 ) ;
#12453=VERTEX_POINT ( 'NONE', #14406 ) ;
#12476=CARTESIAN_POINT ( 'NONE',  ( 0.000000000000000000, 0.000000000000000000, -74.48236190979496030 ) ) ;
#12495=CARTESIAN_POINT ( 'NONE',  ( 0.000000000000000000, -21.99162546567091425, -78.50000000000000000 ) ) ;
#12502=EDGE_LOOP ( 'NONE', ( #14722, #1681, #2502, #12026 ) ) ;
#12552=ORIENTED_EDGE ( 'NONE', *, *, #19039, .T. ) ;
#12559=EDGE_CURVE ( 'NONE', #15541, #5788, #5161, .T. ) ;
#12588=EDGE_LOOP ( 'NONE', ( #7279, #9346 ) ) ;
#12593=UNCERTAINTY_MEASURE_WITH_UNIT (LENGTH_MEASURE( 1.000000000000000082E-05 ), #18657, 'distance_accuracy_value', 'NONE');
#12601=FACE_BOUND ( 'NONE', #19172, .T. ) ;
#12668=TOROIDAL_SURFACE ( 'NONE', #16994, 13.12488928717151637, 5.000000000000000000 ) ;
#12683=EDGE_CURVE ( 'NONE', #12453, #15721, #19595, .T. ) ;
#12685=TOROIDAL_SURFACE ( 'NONE', #19127, 24.63401512838748530, 3.000000000000004441 ) ;
#12688=FACE_OUTER_BOUND ( 'NONE', #20377, .T. ) ;
#12727=DIRECTION ( 'NONE',  ( -0.2588190451025213501, 0.000000000000000000, 0.9659258262890680902 ) ) ;
#12728=EDGE_CURVE ( 'NONE', #21223, #13423, #12013, .T. ) ;
#12750=CARTESIAN_POINT ( 'NONE',  ( 2.100000000000000089, 0.000000000000000000, -126.0000000000000284 ) ) ;
#12840=ADVANCED_FACE ( 'NONE', ( #8310 ), #17057, .F. ) ;
#12860=DIRECTION ( 'NONE',  ( 1.000000000000000000, 0.000000000000000000, 0.000000000000000000 ) ) ;
#12886=CARTESIAN_POINT ( 'NONE',  ( 13.12488928717151637, 1.607335365469798272E-15, -99.99999999999998579 ) ) ;
#12979=DIRECTION ( 'NONE',  ( -1.000000000000000000, 0.000000000000000000, 0.000000000000000000 ) ) ;
#12993=EDGE_CURVE ( 'NONE', #7880, #19741, #199, .T. ) ;
#13016=ORIENTED_EDGE ( 'NONE', *, *, #16549, .T. ) ;
#13066=DIRECTION ( 'NONE',  ( -1.000000000000000000, 1.224646799147352961E-16, 0.000000000000000000 ) ) ;
#13095=DIRECTION ( 'NONE',  ( 0.000000000000000000, 0.000000000000000000, -1.000000000000000000 ) ) ;
#13114=AXIS2_PLACEMENT_3D ( 'NONE', #7375, #14244, #5664 ) ;
#13139=COLOUR_RGB ( '', 0.72549020, 0.75294118, 0.79215686) ;
#13144=DIRECTION ( 'NONE',  ( 0.000000000000000000, 0.000000000000000000, -1.000000000000000000 ) ) ;
#13207=SURFACE_SIDE_STYLE ('',( #6000 ) ) ;
#13352=EDGE_LOOP ( 'NONE', ( #6366, #7049, #21430, #11007 ) ) ;
#13367=DIRECTION ( 'NONE',  ( 1.000000000000000000, 0.000000000000000000, 0.000000000000000000 ) ) ;
#13379=EDGE_LOOP ( 'NONE', ( #20473, #18561, #6712, #17203 ) ) ;
#13413=DIRECTION ( 'NONE',  ( -1.000000000000000000, 0.000000000000000000, 0.000000000000000000 ) ) ;
#13423=VERTEX_POINT ( 'NONE', #9309 ) ;
#13538=ADVANCED_FACE ( 'NONE', ( #4325, #11648 ), #9741, .T. ) ;
#13667=ADVANCED_BREP_SHAPE_REPRESENTATION ( '', ( #21321, #6677 ), #10599 ) ;
#13674=ORIENTED_EDGE ( 'NONE', *, *, #8052, .F. ) ;
#13695=DIRECTION ( 'NONE',  ( 0.000000000000000000, 0.000000000000000000, -1.000000000000000000 ) ) ;
#13704=FILL_AREA_STYLE ('',( #6489 ) ) ;
#13725=ORIENTED_EDGE ( 'NONE', *, *, #5496, .F. ) ;
#13733=CIRCLE ( 'NONE', #16597, 21.80000000000000071 ) ;
#13737=DIRECTION ( 'NONE',  ( -0.000000000000000000, -0.000000000000000000, 1.000000000000000000 ) ) ;
#13744=AXIS2_PLACEMENT_3D ( 'NONE', #20820, #2037, #3385 ) ;
#13755=AXIS2_PLACEMENT_3D ( 'NONE', #15857, #12253, #19219 ) ;
#13827=DIRECTION ( 'NONE',  ( 0.2588190451025213501, -3.169619151431772337E-17, 0.9659258262890680902 ) ) ;
#13852=CIRCLE ( 'NONE', #16017, 2.100000000000000089 ) ;
#13870=CIRCLE ( 'NONE', #8834, 2.100000000000000089 ) ;
#13875=EDGE_CURVE ( 'NONE', #15721, #4133, #11873, .T. ) ;
#13887=CARTESIAN_POINT ( 'NONE',  ( -2.100000000000000089, 2.571758278209441957E-16, -105.0000000000000000 ) ) ;
#13977=EDGE_CURVE ( 'NONE', #21471, #21223, #22114, .T. ) ;
#14016=PRODUCT_DEFINITION ( 'UNKNOWN', '', #939, #656 ) ;
#14023=DIRECTION ( 'NONE',  ( 1.000000000000000000, 0.000000000000000000, 0.000000000000000000 ) ) ;
#14065=ORIENTED_EDGE ( 'NONE', *, *, #16549, .F. ) ;
#14141=EDGE_LOOP ( 'NONE', ( #8632, #7835 ) ) ;
#14149=ORIENTED_EDGE ( 'NONE', *, *, #3156, .T. ) ;
#14163=DIRECTION ( 'NONE',  ( -1.000000000000000000, 0.000000000000000000, 0.000000000000000000 ) ) ;
#14207=DIRECTION ( 'NONE',  ( -0.000000000000000000, -0.000000000000000000, 1.000000000000000000 ) ) ;
#14244=DIRECTION ( 'NONE',  ( -0.000000000000000000, -1.000000000000000000, -0.000000000000000000 ) ) ;
#14260=CIRCLE ( 'NONE', #9225, 25.00000000000001066 ) ;
#14280=DIRECTION ( 'NONE',  ( -0.000000000000000000, -0.000000000000000000, 1.000000000000000000 ) ) ;
#14289=CARTESIAN_POINT ( 'NONE',  ( 0.000000000000000000, 0.000000000000000000, -126.0000000000000284 ) ) ;
#14406=CARTESIAN_POINT ( 'NONE',  ( -4.100000000000000533, 5.021051876504148371E-16, -103.0000000000000000 ) ) ;
#14488=CARTESIAN_POINT ( 'NONE',  ( -23.06814834742187514, 0.000000000000000000, -74.48236190979496030 ) ) ;
#14502=CARTESIAN_POINT ( 'NONE',  ( 13.12488928717151637, 1.903064858314465868E-15, -105.0000000000000000 ) ) ;
#14565=VERTEX_POINT ( 'NONE', #21287 ) ;
#14581=EDGE_CURVE ( 'NONE', #4133, #12432, #9874, .T. ) ;
#14647=CARTESIAN_POINT ( 'NONE',  ( -25.00000000000001066, 0.000000000000000000, -75.00000000000000000 ) ) ;
#14652=DIRECTION ( 'NONE',  ( 1.224646799147353207E-16, 1.000000000000000000, 0.000000000000000000 ) ) ;
#14667=FACE_BOUND ( 'NONE', #14701, .T. ) ;
#14701=EDGE_LOOP ( 'NONE', ( #14149, #1476 ) ) ;
#14722=ORIENTED_EDGE ( 'NONE', *, *, #2230, .F. ) ;
#14777=EDGE_CURVE ( 'NONE', #15721, #12453, #5909, .T. ) ;
#14815=AXIS2_PLACEMENT_3D ( 'NONE', #8266, #6566, #10478 ) ;
#14828=ORIENTED_EDGE ( 'NONE', *, *, #15458, .F. ) ;
#14838=AXIS2_PLACEMENT_3D ( 'NONE', #19233, #15981, #8899 ) ;
#14856=CIRCLE ( 'NONE', #20581, 16.02266676603872142 ) ;
#14871=DIRECTION ( 'NONE',  ( -1.000000000000000000, 0.000000000000000000, 0.000000000000000000 ) ) ;
#14906=VECTOR ( 'NONE', #4661, 1000.000000000000000 ) ;
#14912=EDGE_CURVE ( 'NONE', #15541, #3431, #5557, .T. ) ;
#14988=DIRECTION ( 'NONE',  ( -1.000000000000000000, 0.000000000000000000, 0.000000000000000000 ) ) ;
#14999=CARTESIAN_POINT ( 'NONE',  ( 0.000000000000000000, 0.000000000000000000, -75.00000000000000000 ) ) ;
#15061=( NAMED_UNIT ( * ) PLANE_ANGLE_UNIT ( ) SI_UNIT ( $, .RADIAN. ) );
#15074=CARTESIAN_POINT ( 'NONE',  ( 0.000000000000000000, 0.000000000000000000, -77.51594804401857175 ) ) ;
#15099=CARTESIAN_POINT ( 'NONE',  ( 0.000000000000000000, 0.000000000000000000, -99.99999999999998579 ) ) ;
#15181=EDGE_CURVE ( 'NONE', #8832, #9492, #12042, .T. ) ;
#15192=EDGE_LOOP ( 'NONE', ( #18491, #15557, #543, #19895 ) ) ;
#15243=DIRECTION ( 'NONE',  ( 1.224646799147353207E-16, 1.000000000000000000, 0.000000000000000000 ) ) ;
#15287=DIRECTION ( 'NONE',  ( 0.2588190451025213501, -3.169619151431772337E-17, 0.9659258262890680902 ) ) ;
#15303=CIRCLE ( 'NONE', #4866, 21.99162546567091070 ) ;
#15355=DIRECTION ( 'NONE',  ( -1.000000000000000000, 0.000000000000000000, 0.000000000000000000 ) ) ;
#15397=SURFACE_SIDE_STYLE ('',( #20540 ) ) ;
#15412=ORIENTED_EDGE ( 'NONE', *, *, #7888, .F. ) ;
#15458=EDGE_CURVE ( 'NONE', #21471, #15704, #13852, .T. ) ;
#15536=CIRCLE ( 'NONE', #1148, 5.000000000000000888 ) ;
#15541=VERTEX_POINT ( 'NONE', #5617 ) ;
#15557=ORIENTED_EDGE ( 'NONE', *, *, #19718, .F. ) ;
#15634=ORIENTED_EDGE ( 'NONE', *, *, #3156, .F. ) ;
#15651=DIRECTION ( 'NONE',  ( 1.000000000000000000, 0.000000000000000000, 0.000000000000000000 ) ) ;
#15657=EDGE_LOOP ( 'NONE', ( #4335, #7476 ) ) ;
#15704=VERTEX_POINT ( 'NONE', #5501 ) ;
#15721=VERTEX_POINT ( 'NONE', #342 ) ;
#15741=DIRECTION ( 'NONE',  ( 0.000000000000000000, 0.000000000000000000, -1.000000000000000000 ) ) ;
#15757=ADVANCED_FACE ( 'NONE', ( #12601, #5273 ), #12154, .T. ) ;
#15794=CARTESIAN_POINT ( 'NONE',  ( 0.000000000000000000, 0.000000000000000000, -75.05807060175870049 ) ) ;
#15827=DIRECTION ( 'NONE',  ( 0.000000000000000000, -1.000000000000000000, 0.000000000000000000 ) ) ;
#15849=FACE_OUTER_BOUND ( 'NONE', #20703, .T. ) ;
#15852=ORIENTED_EDGE ( 'NONE', *, *, #989, .T. ) ;
#15857=CARTESIAN_POINT ( 'NONE',  ( 24.63401512838748530, 0.000000000000000000, -77.51594804401857175 ) ) ;
#15892=CIRCLE ( 'NONE', #14815, 21.80000000000000071 ) ;
#15946=AXIS2_PLACEMENT_3D ( 'NONE', #14999, #21612, #11168 ) ;
#15970=EDGE_LOOP ( 'NONE', ( #19870, #13674 ) ) ;
#15981=DIRECTION ( 'NONE',  ( 0.000000000000000000, 0.000000000000000000, -1.000000000000000000 ) ) ;
#16017=AXIS2_PLACEMENT_3D ( 'NONE', #5055, #11931, #18798 ) ;
#16058=APPLICATION_CONTEXT ( 'automotive_design' ) ;
#16072=DIRECTION ( 'NONE',  ( -0.000000000000000000, -0.000000000000000000, 1.000000000000000000 ) ) ;
#16081=FACE_OUTER_BOUND ( 'NONE', #10856, .T. ) ;
#16177=CARTESIAN_POINT ( 'NONE',  ( 0.000000000000000000, 0.000000000000000000, -126.0000000000000284 ) ) ;
#16226=DIRECTION ( 'NONE',  ( 0.000000000000000000, 0.000000000000000000, 1.000000000000000000 ) ) ;
#16255=EDGE_LOOP ( 'NONE', ( #17230, #6482 ) ) ;
#16260=PLANE ( 'NONE',  #5804 ) ;
#16263=AXIS2_PLACEMENT_3D ( 'NONE', #5970, #6187, #2587 ) ;
#16278=AXIS2_PLACEMENT_3D ( 'NONE', #16177, #14280, #17978 ) ;
#16305=CARTESIAN_POINT ( 'NONE',  ( -4.100000000000000533, 5.021051876504148371E-16, -75.00000000000000000 ) ) ;
#16363=FILL_AREA_STYLE_COLOUR ( '', #13139 ) ;
#16377=AXIS2_PLACEMENT_3D ( 'NONE', #15794, #7129, #21057 ) ;
#16522=CARTESIAN_POINT ( 'NONE',  ( 0.000000000000000000, 0.000000000000000000, -101.2940952255125922 ) ) ;
#16549=EDGE_CURVE ( 'NONE', #14565, #9583, #19158, .T. ) ;
#16597=AXIS2_PLACEMENT_3D ( 'NONE', #12170, #14207, #7114 ) ;
#16739=DIRECTION ( 'NONE',  ( 1.000000000000000000, 0.000000000000000000, 0.000000000000000000 ) ) ;
#16754=FACE_OUTER_BOUND ( 'NONE', #13379, .T. ) ;
#16779=DIRECTION ( 'NONE',  ( -1.000000000000000000, 0.000000000000000000, 0.000000000000000000 ) ) ;
#16828=DIRECTION ( 'NONE',  ( -0.000000000000000000, -0.000000000000000000, 1.000000000000000000 ) ) ;
#16854=SHAPE_REPRESENTATION_RELATIONSHIP ( 'NONE' , 'NONE' ,  #3834, #13667 ) ;
#16912=EDGE_LOOP ( 'NONE', ( #20790, #9188, #8974, #20899 ) ) ;
#16966=PRODUCT ( 'Removable  Lid', 'Removable  Lid', '', ( #17856 ) ) ;
#16994=AXIS2_PLACEMENT_3D ( 'NONE', #15099, #21935, #18582 ) ;
#17057=TOROIDAL_SURFACE ( 'NONE', #1599, 13.12488928717151637, 3.000000000000000000 ) ;
#17075=DIRECTION ( 'NONE',  ( -0.000000000000000000, -0.000000000000000000, 1.000000000000000000 ) ) ;
#17096=STYLED_ITEM ( 'NONE', ( #18167 ), #21321 ) ;
#17127=AXIS2_PLACEMENT_3D ( 'NONE', #7566, #4385, #2376 ) ;
#17155=DIRECTION ( 'NONE',  ( -1.224646799147353207E-16, 1.000000000000000000, 0.000000000000000000 ) ) ;
#17203=ORIENTED_EDGE ( 'NONE', *, *, #13875, .F. ) ;
#17230=ORIENTED_EDGE ( 'NONE', *, *, #21099, .T. ) ;
#17350=CONICAL_SURFACE ( 'NONE', #11597, 23.06814834742187514, 0.2617993877991500740 ) ;
#17450=DIRECTION ( 'NONE',  ( -0.000000000000000000, -0.000000000000000000, 1.000000000000000000 ) ) ;
#17465=CIRCLE ( 'NONE', #1273, 17.95451841861686049 ) ;
#17491=AXIS2_PLACEMENT_3D ( 'NONE', #1996, #18693, #3256 ) ;
#17517=CARTESIAN_POINT ( 'NONE',  ( 24.63401512838748530, 0.000000000000000000, -77.51594804401857175 ) ) ;
#17690=CIRCLE ( 'NONE', #13744, 3.000000000000002665 ) ;
#17707=DIRECTION ( 'NONE',  ( -0.000000000000000000, -0.000000000000000000, 1.000000000000000000 ) ) ;
#17756=CARTESIAN_POINT ( 'NONE',  ( 0.000000000000000000, 0.000000000000000000, -75.00000000000000000 ) ) ;
#17760=DIRECTION ( 'NONE',  ( -1.000000000000000000, 0.000000000000000000, 0.000000000000000000 ) ) ;
#17790=ORIENTED_EDGE ( 'NONE', *, *, #19718, .T. ) ;
#17832=DIRECTION ( 'NONE',  ( -0.000000000000000000, -0.000000000000000000, 1.000000000000000000 ) ) ;
#17843=VERTEX_POINT ( 'NONE', #5914 ) ;
#17849=CIRCLE ( 'NONE', #18573, 4.100000000000000533 ) ;
#17854=DIRECTION ( 'NONE',  ( -1.224646799147353207E-16, 1.000000000000000000, 0.000000000000000000 ) ) ;
#17856=PRODUCT_CONTEXT ( 'NONE', #4828, 'mechanical' ) ;
#17878=ORIENTED_EDGE ( 'NONE', *, *, #11148, .T. ) ;
#17920=ADVANCED_FACE ( 'NONE', ( #19637 ), #10567, .F. ) ;
#17978=DIRECTION ( 'NONE',  ( 1.000000000000000000, 0.000000000000000000, 0.000000000000000000 ) ) ;
#17986=DIRECTION ( 'NONE',  ( -1.000000000000000000, 0.000000000000000000, 0.000000000000000000 ) ) ;
#18001=DIRECTION ( 'NONE',  ( 1.000000000000000000, 0.000000000000000000, 0.000000000000000000 ) ) ;
#18028=CARTESIAN_POINT ( 'NONE',  ( 0.000000000000000000, 0.000000000000000000, 0.000000000000000000 ) ) ;
#18110=CARTESIAN_POINT ( 'NONE',  ( -21.99162546567091425, 0.000000000000000000, -78.50000000000000000 ) ) ;
#18158=VERTEX_POINT ( 'NONE', #6245 ) ;
#18165=AXIS2_PLACEMENT_3D ( 'NONE', #18827, #15243, #8491 ) ;
#18167=PRESENTATION_STYLE_ASSIGNMENT (( #11295 ) ) ;
#18177=LINE ( 'NONE', #9621, #5087 ) ;
#18400=ADVANCED_FACE ( 'NONE', ( #7674 ), #20189, .F. ) ;
#18403=ORIENTED_EDGE ( 'NONE', *, *, #7416, .F. ) ;
#18423=ORIENTED_EDGE ( 'NONE', *, *, #6211, .F. ) ;
#18433=EDGE_CURVE ( 'NONE', #6505, #14565, #10508, .T. ) ;
#18465=AXIS2_PLACEMENT_3D ( 'NONE', #15074, #10002, #18880 ) ;
#18491=ORIENTED_EDGE ( 'NONE', *, *, #12993, .F. ) ;
#18498=DIRECTION ( 'NONE',  ( 1.000000000000000000, 0.000000000000000000, 0.000000000000000000 ) ) ;
#18520=CARTESIAN_POINT ( 'NONE',  ( 0.000000000000000000, 0.000000000000000000, -105.0000000000000000 ) ) ;
#18544=SURFACE_STYLE_USAGE ( .BOTH. , #15397 ) ;
#18561=ORIENTED_EDGE ( 'NONE', *, *, #273, .T. ) ;
#18573=AXIS2_PLACEMENT_3D ( 'NONE', #6418, #22175, #14988 ) ;
#18582=DIRECTION ( 'NONE',  ( -1.000000000000000000, 0.000000000000000000, 0.000000000000000000 ) ) ;
#18603=ORIENTED_EDGE ( 'NONE', *, *, #21825, .T. ) ;
#18657=( LENGTH_UNIT ( ) NAMED_UNIT ( * ) SI_UNIT ( .MILLI., .METRE. ) );
#18664=CARTESIAN_POINT ( 'NONE',  ( 0.000000000000000000, 0.000000000000000000, -75.00000000000000000 ) ) ;
#18693=DIRECTION ( 'NONE',  ( -0.000000000000000000, -0.000000000000000000, 1.000000000000000000 ) ) ;
#18753=ADVANCED_FACE ( 'NONE', ( #3250 ), #12685, .T. ) ;
#18773=CIRCLE ( 'NONE', #13755, 3.000000000000002665 ) ;
#18791=CIRCLE ( 'NONE', #22000, 21.63401512838748175 ) ;
#18798=DIRECTION ( 'NONE',  ( -1.000000000000000000, 0.000000000000000000, 0.000000000000000000 ) ) ;
#18827=CARTESIAN_POINT ( 'NONE',  ( -24.63401512838748530, 3.016796777712720900E-15, -77.51594804401857175 ) ) ;
#18871=ADVANCED_FACE ( 'NONE', ( #9917 ), #12668, .T. ) ;
#18880=DIRECTION ( 'NONE',  ( 1.000000000000000000, 0.000000000000000000, 0.000000000000000000 ) ) ;
#18920=ADVANCED_FACE ( 'NONE', ( #5056 ), #6550, .T. ) ;
#18966=EDGE_CURVE ( 'NONE', #9583, #14565, #18791, .T. ) ;
#19039=EDGE_CURVE ( 'NONE', #3431, #2867, #8711, .T. ) ;
#19095=DIRECTION ( 'NONE',  ( -1.000000000000000000, 0.000000000000000000, 0.000000000000000000 ) ) ;
#19127=AXIS2_PLACEMENT_3D ( 'NONE', #21934, #13737, #6413 ) ;
#19157=VECTOR ( 'NONE', #19598, 1000.000000000000000 ) ;
#19158=CIRCLE ( 'NONE', #18465, 21.63401512838748175 ) ;
#19172=EDGE_LOOP ( 'NONE', ( #3749, #15852 ) ) ;
#19219=DIRECTION ( 'NONE',  ( 0.000000000000000000, 0.000000000000000000, -1.000000000000000000 ) ) ;
#19233=CARTESIAN_POINT ( 'NONE',  ( 0.000000000000000000, 0.000000000000000000, -105.0000000000000000 ) ) ;
#19249=CIRCLE ( 'NONE', #9559, 13.12488928717151637 ) ;
#19262=CARTESIAN_POINT ( 'NONE',  ( 22.91388766833460977, -2.807094692329320838E-15, -75.05807060175870049 ) ) ;
#19322=DIRECTION ( 'NONE',  ( -0.000000000000000000, -0.000000000000000000, 1.000000000000000000 ) ) ;
#19342=DIRECTION ( 'NONE',  ( 0.000000000000000000, 0.000000000000000000, -1.000000000000000000 ) ) ;
#19357=TOROIDAL_SURFACE ( 'NONE', #20422, 13.12488928717151637, 5.000000000000000000 ) ;
#19425=AXIS2_PLACEMENT_3D ( 'NONE', #5905, #4427, #4316 ) ;
#19523=VECTOR ( 'NONE', #15287, 1000.000000000000000 ) ;
#19595=CIRCLE ( 'NONE', #5541, 4.100000000000000533 ) ;
#19598=DIRECTION ( 'NONE',  ( -0.000000000000000000, -0.000000000000000000, 1.000000000000000000 ) ) ;
#19627=FACE_OUTER_BOUND ( 'NONE', #8030, .T. ) ;
#19637=FACE_OUTER_BOUND ( 'NONE', #8352, .T. ) ;
#19648=ORIENTED_EDGE ( 'NONE', *, *, #21825, .F. ) ;
#19718=EDGE_CURVE ( 'NONE', #8548, #7880, #14856, .T. ) ;
#19722=( NAMED_UNIT ( * ) SI_UNIT ( $, .STERADIAN. ) SOLID_ANGLE_UNIT ( ) );
#19741=VERTEX_POINT ( 'NONE', #7980 ) ;
#19856=AXIS2_PLACEMENT_3D ( 'NONE', #21293, #21190, #14023 ) ;
#19867=VERTEX_POINT ( 'NONE', #18110 ) ;
#19870=ORIENTED_EDGE ( 'NONE', *, *, #6828, .F. ) ;
#19889=AXIS2_PLACEMENT_3D ( 'NONE', #1540, #2774, #4795 ) ;
#19895=ORIENTED_EDGE ( 'NONE', *, *, #1646, .F. ) ;
#19939=AXIS2_PLACEMENT_3D ( 'NONE', #12495, #19342, #3924 ) ;
#19976=VECTOR ( 'NONE', #9365, 1000.000000000000000 ) ;
#20052=DIRECTION ( 'NONE',  ( -0.000000000000000000, -0.000000000000000000, 1.000000000000000000 ) ) ;
#20066=CIRCLE ( 'NONE', #8941, 22.92944763917984474 ) ;
#20189=CONICAL_SURFACE ( 'NONE', #16263, 23.06814834742187514, 0.2617993877991500740 ) ;
#20377=EDGE_LOOP ( 'NONE', ( #9507, #9305, #21582, #18403 ) ) ;
#20422=AXIS2_PLACEMENT_3D ( 'NONE', #20531, #13695, #10204 ) ;
#20473=ORIENTED_EDGE ( 'NONE', *, *, #14777, .T. ) ;
#20506=ADVANCED_FACE ( 'NONE', ( #16754 ), #6501, .T. ) ;
#20531=CARTESIAN_POINT ( 'NONE',  ( 0.000000000000000000, 0.000000000000000000, -99.99999999999998579 ) ) ;
#20540=SURFACE_STYLE_FILL_AREA ( #13704 ) ;
#20580=CONICAL_SURFACE ( 'NONE', #10899, 23.06814834742187514, 0.2617993877991500740 ) ;
#20581=AXIS2_PLACEMENT_3D ( 'NONE', #21464, #1105, #18001 ) ;
#20703=EDGE_LOOP ( 'NONE', ( #5039, #2135, #20811, #15412 ) ) ;
#20790=ORIENTED_EDGE ( 'NONE', *, *, #18966, .F. ) ;
#20796=AXIS2_PLACEMENT_3D ( 'NONE', #14289, #21122, #650 ) ;
#20811=ORIENTED_EDGE ( 'NONE', *, *, #13875, .T. ) ;
#20820=CARTESIAN_POINT ( 'NONE',  ( -13.12488928717151637, 0.000000000000000000, -99.99999999999998579 ) ) ;
#20845=CLOSED_SHELL ( 'NONE', ( #9418, #18753, #18920, #20506, #17920, #8663, #2572, #3447, #186, #8611, #18400, #11272, #11071, #13538, #9907, #18871, #5396, #10381, #4521, #12840, #8578, #7367, #15757 ) ) ;
#20899=ORIENTED_EDGE ( 'NONE', *, *, #18433, .T. ) ;
#20973=AXIS2_PLACEMENT_3D ( 'NONE', #11671, #13144, #3108 ) ;
#21008=EDGE_LOOP ( 'NONE', ( #10891, #10872, #21672, #21363 ) ) ;
#21057=DIRECTION ( 'NONE',  ( -1.000000000000000000, 0.000000000000000000, 0.000000000000000000 ) ) ;
#21099=EDGE_CURVE ( 'NONE', #19867, #19741, #15303, .T. ) ;
#21122=DIRECTION ( 'NONE',  ( -0.000000000000000000, -0.000000000000000000, 1.000000000000000000 ) ) ;
#21188=EDGE_CURVE ( 'NONE', #5788, #15541, #17465, .T. ) ;
#21190=DIRECTION ( 'NONE',  ( -0.000000000000000000, -0.000000000000000000, 1.000000000000000000 ) ) ;
#21200=CARTESIAN_POINT ( 'NONE',  ( 0.000000000000000000, 0.000000000000000000, -75.00000000000000000 ) ) ;
#21223=VERTEX_POINT ( 'NONE', #7704 ) ;
#21277=LINE ( 'NONE', #12750, #19157 ) ;
#21287=CARTESIAN_POINT ( 'NONE',  ( -21.63401512838748175, 2.649402737968514273E-15, -77.51594804401857175 ) ) ;
#21293=CARTESIAN_POINT ( 'NONE',  ( 0.000000000000000000, 0.000000000000000000, -126.0000000000000284 ) ) ;
#21321=MANIFOLD_SOLID_BREP ( 'Revolve1', #20845 ) ;
#21363=ORIENTED_EDGE ( 'NONE', *, *, #6828, .T. ) ;
#21365=DIRECTION ( 'NONE',  ( -1.000000000000000000, 0.000000000000000000, 0.000000000000000000 ) ) ;
#21430=ORIENTED_EDGE ( 'NONE', *, *, #19039, .F. ) ;
#21464=CARTESIAN_POINT ( 'NONE',  ( 0.000000000000000000, 0.000000000000000000, -100.7764571353075524 ) ) ;
#21471=VERTEX_POINT ( 'NONE', #13887 ) ;
#21485=EDGE_CURVE ( 'NONE', #15704, #21471, #13870, .T. ) ;
#21582=ORIENTED_EDGE ( 'NONE', *, *, #21099, .F. ) ;
#21612=DIRECTION ( 'NONE',  ( 0.000000000000000000, 0.000000000000000000, -1.000000000000000000 ) ) ;
#21637=FACE_OUTER_BOUND ( 'NONE', #3264, .T. ) ;
#21657=AXIS2_PLACEMENT_3D ( 'NONE', #1368, #4732, #12860 ) ;
#21672=ORIENTED_EDGE ( 'NONE', *, *, #1440, .T. ) ;
#21698=DIRECTION ( 'NONE',  ( 0.000000000000000000, 0.000000000000000000, -1.000000000000000000 ) ) ;
#21727=PLANE ( 'NONE',  #15946 ) ;
#21773=EDGE_CURVE ( 'NONE', #14565, #18158, #5580, .T. ) ;
#21790=FACE_OUTER_BOUND ( 'NONE', #12588, .T. ) ;
#21791=UNCERTAINTY_MEASURE_WITH_UNIT (LENGTH_MEASURE( 1.000000000000000082E-05 ), #11184, 'distance_accuracy_value', 'NONE');
#21792=CARTESIAN_POINT ( 'NONE',  ( -22.91388766833460977, 0.000000000000000000, -75.05807060175870049 ) ) ;
#21798=CARTESIAN_POINT ( 'NONE',  ( 0.000000000000000000, 0.000000000000000000, -99.99999999999998579 ) ) ;
#21825=EDGE_CURVE ( 'NONE', #1266, #17843, #19249, .T. ) ;
#21899=FACE_BOUND ( 'NONE', #15657, .T. ) ;
#21934=CARTESIAN_POINT ( 'NONE',  ( 0.000000000000000000, 0.000000000000000000, -77.51594804401857175 ) ) ;
#21935=DIRECTION ( 'NONE',  ( 0.000000000000000000, 0.000000000000000000, -1.000000000000000000 ) ) ;
#21956=ORIENTED_EDGE ( 'NONE', *, *, #1440, .F. ) ;
#22000=AXIS2_PLACEMENT_3D ( 'NONE', #1906, #3589, #15651 ) ;
#22024=CARTESIAN_POINT ( 'NONE',  ( 0.000000000000000000, 0.000000000000000000, -103.0000000000000000 ) ) ;
#22032=ORIENTED_EDGE ( 'NONE', *, *, #2399, .F. ) ;
#22062=EDGE_CURVE ( 'NONE', #6505, #7331, #7780, .T. ) ;
#22088=CARTESIAN_POINT ( 'NONE',  ( 0.000000000000000000, 0.000000000000000000, -103.0000000000000000 ) ) ;
#22114=LINE ( 'NONE', #11768, #14906 ) ;
#22133=DIRECTION ( 'NONE',  ( -1.000000000000000000, 0.000000000000000000, 0.000000000000000000 ) ) ;
#22137=( NAMED_UNIT ( * ) PLANE_ANGLE_UNIT ( ) SI_UNIT ( $, .RADIAN. ) );
#22142=DIRECTION ( 'NONE',  ( -0.000000000000000000, -0.000000000000000000, 1.000000000000000000 ) ) ;
#22175=DIRECTION ( 'NONE',  ( -0.000000000000000000, -0.000000000000000000, 1.000000000000000000 ) ) ;
#22202=CARTESIAN_POINT ( 'NONE',  ( 0.000000000000000000, 0.000000000000000000, -105.0000000000000000 ) ) ;
#22249=DIRECTION ( 'NONE',  ( -1.000000000000000000, 0.000000000000000000, 0.000000000000000000 ) ) ;
ENDSEC;
END-ISO-10303-21;
